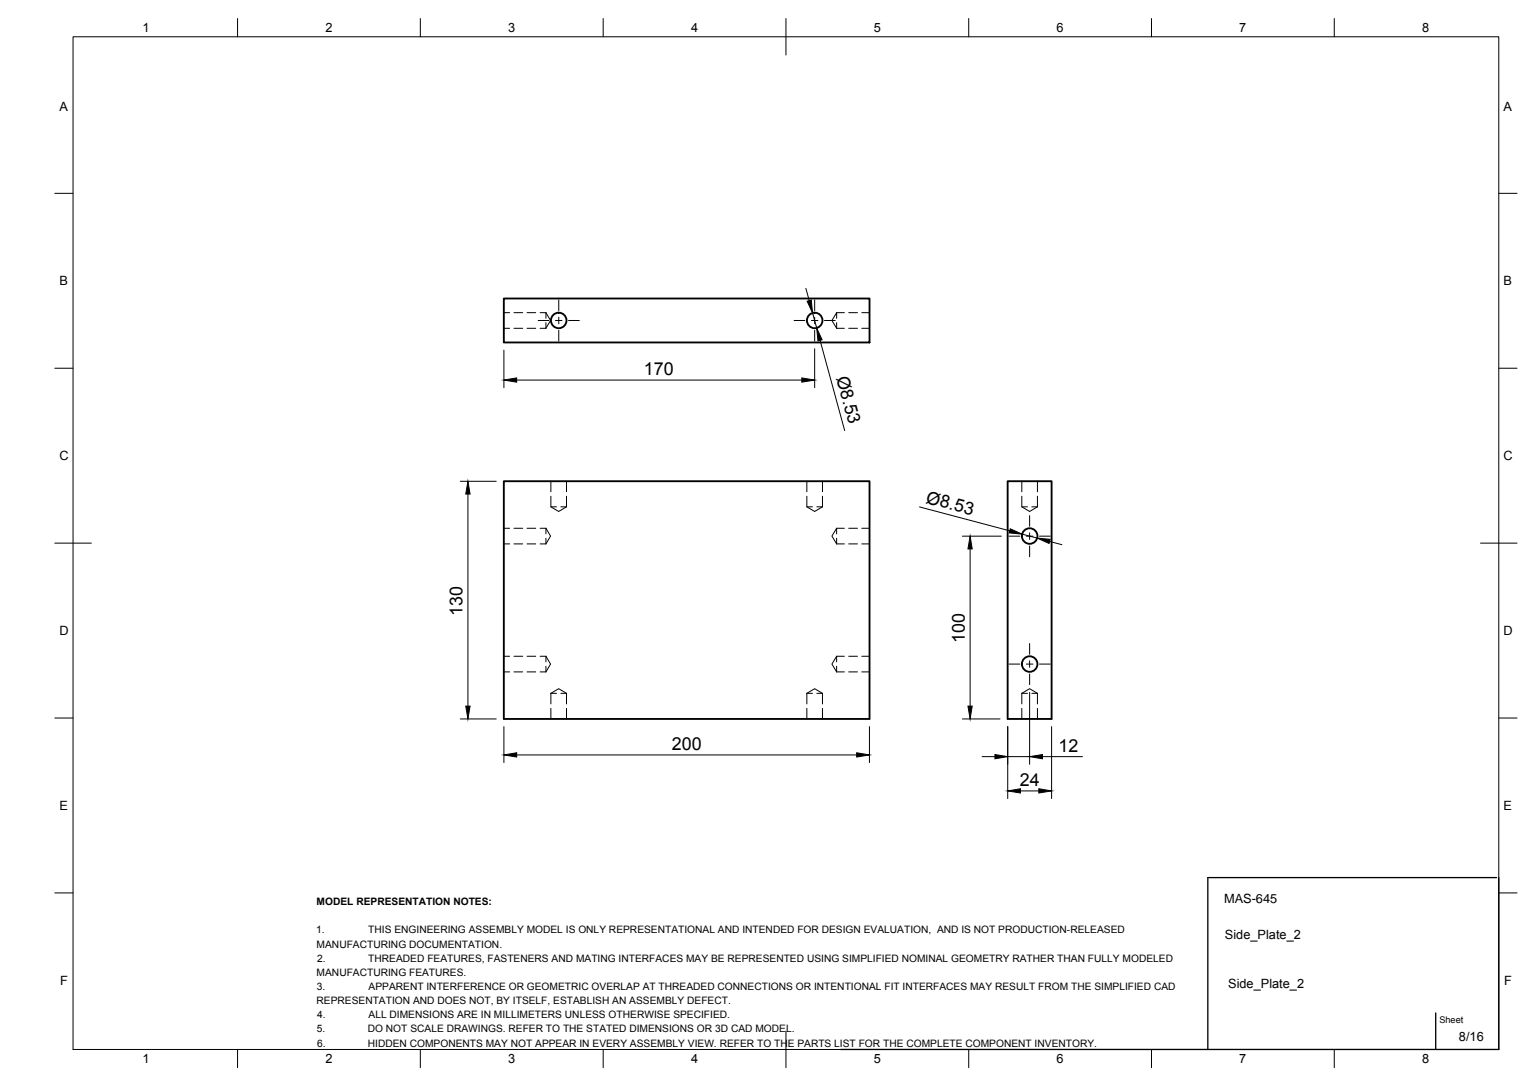
ISO-10303-21;
HEADER;
FILE_DESCRIPTION((''),'2;1');
FILE_NAME('Side_Plate_2.step','2026-10-09T10:54:55-07:00',(''),(''),'','','');
FILE_SCHEMA (('AUTOMOTIVE_DESIGN { 1 0 10303 214 3 1 1 }'));
ENDSEC;
DATA;
#10=MECHANICAL_DESIGN_GEOMETRIC_PRESENTATION_REPRESENTATION('',(#599),#63824);
#569=SHAPE_REPRESENTATION_RELATIONSHIP('SRR','None',#63883,#584) ;
#584=ADVANCED_BREP_SHAPE_REPRESENTATION('',(#614),#63813) ;
#599=STYLED_ITEM('',(#63963),#614) ;
#614=MANIFOLD_SOLID_BREP('Body1',#15498) ;
#723=FACE_BOUND('',#2671,.T.) ;
#724=FACE_BOUND('',#2672,.T.) ;
#725=FACE_BOUND('',#2679,.T.) ;
#726=FACE_BOUND('',#2680,.T.) ;
#727=FACE_BOUND('',#2683,.T.) ;
#728=FACE_BOUND('',#2684,.T.) ;
#729=FACE_BOUND('',#2686,.T.) ;
#730=FACE_BOUND('',#2687,.T.) ;
#876=PLANE('',#16011) ;
#877=PLANE('',#16020) ;
#878=PLANE('',#16021) ;
#879=PLANE('',#16022) ;
#880=PLANE('',#16023) ;
#881=PLANE('',#16024) ;
#1192=CYLINDRICAL_SURFACE('',#15989,4.263) ;
#1193=CYLINDRICAL_SURFACE('',#15993,4.263) ;
#1194=CYLINDRICAL_SURFACE('',#15997,4.263) ;
#1195=CYLINDRICAL_SURFACE('',#16001,4.263) ;
#1196=CYLINDRICAL_SURFACE('',#16005,4.263) ;
#1197=CYLINDRICAL_SURFACE('',#16009,4.263) ;
#1198=CYLINDRICAL_SURFACE('',#16014,4.263) ;
#1199=CYLINDRICAL_SURFACE('',#16018,4.263) ;
#1699=FACE_OUTER_BOUND('',#2658,.T.) ;
#1700=FACE_OUTER_BOUND('',#2659,.T.) ;
#1701=FACE_OUTER_BOUND('',#2660,.T.) ;
#1702=FACE_OUTER_BOUND('',#2661,.T.) ;
#1703=FACE_OUTER_BOUND('',#2662,.T.) ;
#1704=FACE_OUTER_BOUND('',#2663,.T.) ;
#1705=FACE_OUTER_BOUND('',#2664,.T.) ;
#1706=FACE_OUTER_BOUND('',#2665,.T.) ;
#1707=FACE_OUTER_BOUND('',#2666,.T.) ;
#1708=FACE_OUTER_BOUND('',#2667,.T.) ;
#1709=FACE_OUTER_BOUND('',#2668,.T.) ;
#1710=FACE_OUTER_BOUND('',#2669,.T.) ;
#1711=FACE_OUTER_BOUND('',#2670,.T.) ;
#1712=FACE_OUTER_BOUND('',#2673,.T.) ;
#1713=FACE_OUTER_BOUND('',#2674,.T.) ;
#1714=FACE_OUTER_BOUND('',#2675,.T.) ;
#1715=FACE_OUTER_BOUND('',#2676,.T.) ;
#1716=FACE_OUTER_BOUND('',#2677,.T.) ;
#1717=FACE_OUTER_BOUND('',#2678,.T.) ;
#1718=FACE_OUTER_BOUND('',#2681,.T.) ;
#1719=FACE_OUTER_BOUND('',#2682,.T.) ;
#1720=FACE_OUTER_BOUND('',#2685,.T.) ;
#2658=EDGE_LOOP('',(#10422,#10423,#10424)) ;
#2659=EDGE_LOOP('',(#10425,#10426,#10427,#10428)) ;
#2660=EDGE_LOOP('',(#10429,#10430,#10431)) ;
#2661=EDGE_LOOP('',(#10432,#10433,#10434,#10435)) ;
#2662=EDGE_LOOP('',(#10436,#10437,#10438)) ;
#2663=EDGE_LOOP('',(#10439,#10440,#10441,#10442)) ;
#2664=EDGE_LOOP('',(#10443,#10444,#10445)) ;
#2665=EDGE_LOOP('',(#10446,#10447,#10448,#10449)) ;
#2666=EDGE_LOOP('',(#10450,#10451,#10452)) ;
#2667=EDGE_LOOP('',(#10453,#10454,#10455,#10456)) ;
#2668=EDGE_LOOP('',(#10457,#10458,#10459)) ;
#2669=EDGE_LOOP('',(#10460,#10461,#10462,#10463)) ;
#2670=EDGE_LOOP('',(#10464,#10465,#10466,#10467)) ;
#2671=EDGE_LOOP('',(#10468)) ;
#2672=EDGE_LOOP('',(#10469)) ;
#2673=EDGE_LOOP('',(#10470,#10471,#10472)) ;
#2674=EDGE_LOOP('',(#10473,#10474,#10475,#10476)) ;
#2675=EDGE_LOOP('',(#10477,#10478,#10479)) ;
#2676=EDGE_LOOP('',(#10480,#10481,#10482,#10483)) ;
#2677=EDGE_LOOP('',(#10484,#10485,#10486,#10487)) ;
#2678=EDGE_LOOP('',(#10488,#10489,#10490,#10491)) ;
#2679=EDGE_LOOP('',(#10492)) ;
#2680=EDGE_LOOP('',(#10493)) ;
#2681=EDGE_LOOP('',(#10494,#10495,#10496,#10497)) ;
#2682=EDGE_LOOP('',(#10498,#10499,#10500,#10501)) ;
#2683=EDGE_LOOP('',(#10502)) ;
#2684=EDGE_LOOP('',(#10503)) ;
#2685=EDGE_LOOP('',(#10504,#10505,#10506,#10507)) ;
#2686=EDGE_LOOP('',(#10508)) ;
#2687=EDGE_LOOP('',(#10509)) ;
#3626=CIRCLE('',#15988,4.263) ;
#3627=CIRCLE('',#15990,4.263) ;
#3628=CIRCLE('',#15992,4.263) ;
#3629=CIRCLE('',#15994,4.263) ;
#3630=CIRCLE('',#15996,4.263) ;
#3631=CIRCLE('',#15998,4.263) ;
#3632=CIRCLE('',#16000,4.263) ;
#3633=CIRCLE('',#16002,4.263) ;
#3634=CIRCLE('',#16004,4.263) ;
#3635=CIRCLE('',#16006,4.263) ;
#3636=CIRCLE('',#16008,4.263) ;
#3637=CIRCLE('',#16010,4.263) ;
#3638=CIRCLE('',#16013,4.263) ;
#3639=CIRCLE('',#16015,4.263) ;
#3640=CIRCLE('',#16017,4.263) ;
#3641=CIRCLE('',#16019,4.263) ;
#4848=LINE('',#23703,#5504) ;
#4849=LINE('',#23708,#5505) ;
#4850=LINE('',#23712,#5506) ;
#4851=LINE('',#23717,#5507) ;
#4852=LINE('',#23721,#5508) ;
#4853=LINE('',#23726,#5509) ;
#4854=LINE('',#23730,#5510) ;
#4855=LINE('',#23735,#5511) ;
#4856=LINE('',#23739,#5512) ;
#4857=LINE('',#23744,#5513) ;
#4858=LINE('',#23748,#5514) ;
#4859=LINE('',#23753,#5515) ;
#4860=LINE('',#23757,#5516) ;
#4861=LINE('',#23759,#5517) ;
#4862=LINE('',#23761,#5518) ;
#4863=LINE('',#23762,#5519) ;
#4864=LINE('',#23766,#5520) ;
#4865=LINE('',#23770,#5521) ;
#4866=LINE('',#23775,#5522) ;
#4867=LINE('',#23779,#5523) ;
#4868=LINE('',#23784,#5524) ;
#4869=LINE('',#23785,#5525) ;
#4870=LINE('',#23786,#5526) ;
#4871=LINE('',#23789,#5527) ;
#4872=LINE('',#23790,#5528) ;
#4873=LINE('',#23793,#5529) ;
#4874=LINE('',#23794,#5530) ;
#4875=LINE('',#23796,#5531) ;
#5504=VECTOR('',#18686,2.42186816158307) ;
#5505=VECTOR('',#18693,4.263) ;
#5506=VECTOR('',#18696,2.42186816158307) ;
#5507=VECTOR('',#18703,4.263) ;
#5508=VECTOR('',#18706,2.42186816158307) ;
#5509=VECTOR('',#18713,4.263) ;
#5510=VECTOR('',#18716,2.42186816158307) ;
#5511=VECTOR('',#18723,4.263) ;
#5512=VECTOR('',#18726,2.42186816158307) ;
#5513=VECTOR('',#18733,4.263) ;
#5514=VECTOR('',#18736,2.42186816158307) ;
#5515=VECTOR('',#18743,4.263) ;
#5516=VECTOR('',#18746,10.) ;
#5517=VECTOR('',#18747,10.) ;
#5518=VECTOR('',#18748,10.) ;
#5519=VECTOR('',#18749,10.) ;
#5520=VECTOR('',#18752,2.42186816158307) ;
#5521=VECTOR('',#18757,4.263) ;
#5522=VECTOR('',#18762,2.42186816158307) ;
#5523=VECTOR('',#18767,4.263) ;
#5524=VECTOR('',#18772,10.) ;
#5525=VECTOR('',#18773,10.) ;
#5526=VECTOR('',#18774,10.) ;
#5527=VECTOR('',#18777,10.) ;
#5528=VECTOR('',#18778,10.) ;
#5529=VECTOR('',#18781,10.) ;
#5530=VECTOR('',#18782,10.) ;
#5531=VECTOR('',#18785,10.) ;
#6220=VERTEX_POINT('',#23701) ;
#6221=VERTEX_POINT('',#23702) ;
#6222=VERTEX_POINT('',#23706) ;
#6223=VERTEX_POINT('',#23710) ;
#6224=VERTEX_POINT('',#23711) ;
#6225=VERTEX_POINT('',#23715) ;
#6226=VERTEX_POINT('',#23719) ;
#6227=VERTEX_POINT('',#23720) ;
#6228=VERTEX_POINT('',#23724) ;
#6229=VERTEX_POINT('',#23728) ;
#6230=VERTEX_POINT('',#23729) ;
#6231=VERTEX_POINT('',#23733) ;
#6232=VERTEX_POINT('',#23737) ;
#6233=VERTEX_POINT('',#23738) ;
#6234=VERTEX_POINT('',#23742) ;
#6235=VERTEX_POINT('',#23746) ;
#6236=VERTEX_POINT('',#23747) ;
#6237=VERTEX_POINT('',#23751) ;
#6238=VERTEX_POINT('',#23755) ;
#6239=VERTEX_POINT('',#23756) ;
#6240=VERTEX_POINT('',#23758) ;
#6241=VERTEX_POINT('',#23760) ;
#6242=VERTEX_POINT('',#23764) ;
#6243=VERTEX_POINT('',#23765) ;
#6244=VERTEX_POINT('',#23769) ;
#6245=VERTEX_POINT('',#23773) ;
#6246=VERTEX_POINT('',#23774) ;
#6247=VERTEX_POINT('',#23778) ;
#6248=VERTEX_POINT('',#23782) ;
#6249=VERTEX_POINT('',#23783) ;
#6250=VERTEX_POINT('',#23788) ;
#6251=VERTEX_POINT('',#23792) ;
#7765=EDGE_CURVE('',#6220,#6221,#4848,.T.) ;
#7766=EDGE_CURVE('',#6221,#6221,#3626,.T.) ;
#7767=EDGE_CURVE('',#6222,#6222,#3627,.T.) ;
#7768=EDGE_CURVE('',#6222,#6221,#4849,.T.) ;
#7769=EDGE_CURVE('',#6223,#6224,#4850,.T.) ;
#7770=EDGE_CURVE('',#6224,#6224,#3628,.T.) ;
#7771=EDGE_CURVE('',#6225,#6225,#3629,.T.) ;
#7772=EDGE_CURVE('',#6225,#6224,#4851,.T.) ;
#7773=EDGE_CURVE('',#6226,#6227,#4852,.T.) ;
#7774=EDGE_CURVE('',#6227,#6227,#3630,.T.) ;
#7775=EDGE_CURVE('',#6228,#6228,#3631,.T.) ;
#7776=EDGE_CURVE('',#6228,#6227,#4853,.T.) ;
#7777=EDGE_CURVE('',#6229,#6230,#4854,.T.) ;
#7778=EDGE_CURVE('',#6230,#6230,#3632,.T.) ;
#7779=EDGE_CURVE('',#6231,#6231,#3633,.T.) ;
#7780=EDGE_CURVE('',#6231,#6230,#4855,.T.) ;
#7781=EDGE_CURVE('',#6232,#6233,#4856,.T.) ;
#7782=EDGE_CURVE('',#6233,#6233,#3634,.T.) ;
#7783=EDGE_CURVE('',#6234,#6234,#3635,.F.) ;
#7784=EDGE_CURVE('',#6234,#6233,#4857,.T.) ;
#7785=EDGE_CURVE('',#6235,#6236,#4858,.T.) ;
#7786=EDGE_CURVE('',#6236,#6236,#3636,.T.) ;
#7787=EDGE_CURVE('',#6237,#6237,#3637,.F.) ;
#7788=EDGE_CURVE('',#6237,#6236,#4859,.T.) ;
#7789=EDGE_CURVE('',#6238,#6239,#4860,.T.) ;
#7790=EDGE_CURVE('',#6239,#6240,#4861,.T.) ;
#7791=EDGE_CURVE('',#6240,#6241,#4862,.T.) ;
#7792=EDGE_CURVE('',#6241,#6238,#4863,.T.) ;
#7793=EDGE_CURVE('',#6242,#6243,#4864,.T.) ;
#7794=EDGE_CURVE('',#6243,#6243,#3638,.T.) ;
#7795=EDGE_CURVE('',#6243,#6244,#4865,.T.) ;
#7796=EDGE_CURVE('',#6244,#6244,#3639,.F.) ;
#7797=EDGE_CURVE('',#6245,#6246,#4866,.T.) ;
#7798=EDGE_CURVE('',#6246,#6246,#3640,.T.) ;
#7799=EDGE_CURVE('',#6246,#6247,#4867,.T.) ;
#7800=EDGE_CURVE('',#6247,#6247,#3641,.F.) ;
#7801=EDGE_CURVE('',#6248,#6249,#4868,.T.) ;
#7802=EDGE_CURVE('',#6249,#6240,#4869,.T.) ;
#7803=EDGE_CURVE('',#6248,#6239,#4870,.T.) ;
#7804=EDGE_CURVE('',#6249,#6250,#4871,.T.) ;
#7805=EDGE_CURVE('',#6250,#6241,#4872,.T.) ;
#7806=EDGE_CURVE('',#6250,#6251,#4873,.T.) ;
#7807=EDGE_CURVE('',#6251,#6238,#4874,.T.) ;
#7808=EDGE_CURVE('',#6251,#6248,#4875,.T.) ;
#10422=ORIENTED_EDGE('',*,*,#7765,.T.) ;
#10423=ORIENTED_EDGE('',*,*,#7766,.F.) ;
#10424=ORIENTED_EDGE('',*,*,#7765,.F.) ;
#10425=ORIENTED_EDGE('',*,*,#7767,.F.) ;
#10426=ORIENTED_EDGE('',*,*,#7768,.T.) ;
#10427=ORIENTED_EDGE('',*,*,#7766,.T.) ;
#10428=ORIENTED_EDGE('',*,*,#7768,.F.) ;
#10429=ORIENTED_EDGE('',*,*,#7769,.T.) ;
#10430=ORIENTED_EDGE('',*,*,#7770,.F.) ;
#10431=ORIENTED_EDGE('',*,*,#7769,.F.) ;
#10432=ORIENTED_EDGE('',*,*,#7771,.F.) ;
#10433=ORIENTED_EDGE('',*,*,#7772,.T.) ;
#10434=ORIENTED_EDGE('',*,*,#7770,.T.) ;
#10435=ORIENTED_EDGE('',*,*,#7772,.F.) ;
#10436=ORIENTED_EDGE('',*,*,#7773,.T.) ;
#10437=ORIENTED_EDGE('',*,*,#7774,.F.) ;
#10438=ORIENTED_EDGE('',*,*,#7773,.F.) ;
#10439=ORIENTED_EDGE('',*,*,#7775,.F.) ;
#10440=ORIENTED_EDGE('',*,*,#7776,.T.) ;
#10441=ORIENTED_EDGE('',*,*,#7774,.T.) ;
#10442=ORIENTED_EDGE('',*,*,#7776,.F.) ;
#10443=ORIENTED_EDGE('',*,*,#7777,.T.) ;
#10444=ORIENTED_EDGE('',*,*,#7778,.F.) ;
#10445=ORIENTED_EDGE('',*,*,#7777,.F.) ;
#10446=ORIENTED_EDGE('',*,*,#7779,.F.) ;
#10447=ORIENTED_EDGE('',*,*,#7780,.T.) ;
#10448=ORIENTED_EDGE('',*,*,#7778,.T.) ;
#10449=ORIENTED_EDGE('',*,*,#7780,.F.) ;
#10450=ORIENTED_EDGE('',*,*,#7781,.T.) ;
#10451=ORIENTED_EDGE('',*,*,#7782,.F.) ;
#10452=ORIENTED_EDGE('',*,*,#7781,.F.) ;
#10453=ORIENTED_EDGE('',*,*,#7783,.F.) ;
#10454=ORIENTED_EDGE('',*,*,#7784,.T.) ;
#10455=ORIENTED_EDGE('',*,*,#7782,.T.) ;
#10456=ORIENTED_EDGE('',*,*,#7784,.F.) ;
#10457=ORIENTED_EDGE('',*,*,#7785,.T.) ;
#10458=ORIENTED_EDGE('',*,*,#7786,.F.) ;
#10459=ORIENTED_EDGE('',*,*,#7785,.F.) ;
#10460=ORIENTED_EDGE('',*,*,#7787,.F.) ;
#10461=ORIENTED_EDGE('',*,*,#7788,.T.) ;
#10462=ORIENTED_EDGE('',*,*,#7786,.T.) ;
#10463=ORIENTED_EDGE('',*,*,#7788,.F.) ;
#10464=ORIENTED_EDGE('',*,*,#7789,.T.) ;
#10465=ORIENTED_EDGE('',*,*,#7790,.T.) ;
#10466=ORIENTED_EDGE('',*,*,#7791,.T.) ;
#10467=ORIENTED_EDGE('',*,*,#7792,.T.) ;
#10468=ORIENTED_EDGE('',*,*,#7783,.T.) ;
#10469=ORIENTED_EDGE('',*,*,#7787,.T.) ;
#10470=ORIENTED_EDGE('',*,*,#7793,.T.) ;
#10471=ORIENTED_EDGE('',*,*,#7794,.T.) ;
#10472=ORIENTED_EDGE('',*,*,#7793,.F.) ;
#10473=ORIENTED_EDGE('',*,*,#7794,.F.) ;
#10474=ORIENTED_EDGE('',*,*,#7795,.T.) ;
#10475=ORIENTED_EDGE('',*,*,#7796,.T.) ;
#10476=ORIENTED_EDGE('',*,*,#7795,.F.) ;
#10477=ORIENTED_EDGE('',*,*,#7797,.T.) ;
#10478=ORIENTED_EDGE('',*,*,#7798,.T.) ;
#10479=ORIENTED_EDGE('',*,*,#7797,.F.) ;
#10480=ORIENTED_EDGE('',*,*,#7798,.F.) ;
#10481=ORIENTED_EDGE('',*,*,#7799,.T.) ;
#10482=ORIENTED_EDGE('',*,*,#7800,.T.) ;
#10483=ORIENTED_EDGE('',*,*,#7799,.F.) ;
#10484=ORIENTED_EDGE('',*,*,#7801,.T.) ;
#10485=ORIENTED_EDGE('',*,*,#7802,.T.) ;
#10486=ORIENTED_EDGE('',*,*,#7790,.F.) ;
#10487=ORIENTED_EDGE('',*,*,#7803,.F.) ;
#10488=ORIENTED_EDGE('',*,*,#7804,.T.) ;
#10489=ORIENTED_EDGE('',*,*,#7805,.T.) ;
#10490=ORIENTED_EDGE('',*,*,#7791,.F.) ;
#10491=ORIENTED_EDGE('',*,*,#7802,.F.) ;
#10492=ORIENTED_EDGE('',*,*,#7767,.T.) ;
#10493=ORIENTED_EDGE('',*,*,#7771,.T.) ;
#10494=ORIENTED_EDGE('',*,*,#7806,.T.) ;
#10495=ORIENTED_EDGE('',*,*,#7807,.T.) ;
#10496=ORIENTED_EDGE('',*,*,#7792,.F.) ;
#10497=ORIENTED_EDGE('',*,*,#7805,.F.) ;
#10498=ORIENTED_EDGE('',*,*,#7808,.T.) ;
#10499=ORIENTED_EDGE('',*,*,#7803,.T.) ;
#10500=ORIENTED_EDGE('',*,*,#7789,.F.) ;
#10501=ORIENTED_EDGE('',*,*,#7807,.F.) ;
#10502=ORIENTED_EDGE('',*,*,#7775,.T.) ;
#10503=ORIENTED_EDGE('',*,*,#7779,.T.) ;
#10504=ORIENTED_EDGE('',*,*,#7808,.F.) ;
#10505=ORIENTED_EDGE('',*,*,#7806,.F.) ;
#10506=ORIENTED_EDGE('',*,*,#7804,.F.) ;
#10507=ORIENTED_EDGE('',*,*,#7801,.F.) ;
#10508=ORIENTED_EDGE('',*,*,#7796,.F.) ;
#10509=ORIENTED_EDGE('',*,*,#7800,.F.) ;
#14530=CONICAL_SURFACE('',#15987,2.42186816158307,1.02974425867665) ;
#14531=CONICAL_SURFACE('',#15991,2.42186816158307,1.02974425867665) ;
#14532=CONICAL_SURFACE('',#15995,2.42186816158307,1.02974425867665) ;
#14533=CONICAL_SURFACE('',#15999,2.42186816158307,1.02974425867665) ;
#14534=CONICAL_SURFACE('',#16003,2.42186816158307,1.02974425867665) ;
#14535=CONICAL_SURFACE('',#16007,2.42186816158307,1.02974425867665) ;
#14536=CONICAL_SURFACE('',#16012,2.42186816158307,1.02974425867665) ;
#14537=CONICAL_SURFACE('',#16016,2.42186816158307,1.02974425867665) ;
#14787=ADVANCED_FACE('',(#1699),#14530,.F.) ;
#14788=ADVANCED_FACE('',(#1700),#1192,.F.) ;
#14789=ADVANCED_FACE('',(#1701),#14531,.F.) ;
#14790=ADVANCED_FACE('',(#1702),#1193,.F.) ;
#14791=ADVANCED_FACE('',(#1703),#14532,.F.) ;
#14792=ADVANCED_FACE('',(#1704),#1194,.F.) ;
#14793=ADVANCED_FACE('',(#1705),#14533,.F.) ;
#14794=ADVANCED_FACE('',(#1706),#1195,.F.) ;
#14795=ADVANCED_FACE('',(#1707),#14534,.F.) ;
#14796=ADVANCED_FACE('',(#1708),#1196,.F.) ;
#14797=ADVANCED_FACE('',(#1709),#14535,.F.) ;
#14798=ADVANCED_FACE('',(#1710),#1197,.F.) ;
#14799=ADVANCED_FACE('',(#1711,#723,#724),#876,.F.) ;
#14800=ADVANCED_FACE('',(#1712),#14536,.F.) ;
#14801=ADVANCED_FACE('',(#1713),#1198,.F.) ;
#14802=ADVANCED_FACE('',(#1714),#14537,.F.) ;
#14803=ADVANCED_FACE('',(#1715),#1199,.F.) ;
#14804=ADVANCED_FACE('',(#1716),#877,.F.) ;
#14805=ADVANCED_FACE('',(#1717,#725,#726),#878,.F.) ;
#14806=ADVANCED_FACE('',(#1718),#879,.F.) ;
#14807=ADVANCED_FACE('',(#1719,#727,#728),#880,.F.) ;
#14808=ADVANCED_FACE('',(#1720,#729,#730),#881,.T.) ;
#15498=CLOSED_SHELL('',(#14787,#14788,#14789,#14790,#14791,#14792,#14793,
#14794,#14795,#14796,#14797,#14798,#14799,#14800,#14801,#14802,#14803,#14804,
#14805,#14806,#14807,#14808)) ;
#15986=AXIS2_PLACEMENT_3D('',#23699,#18682,#18683) ;
#15987=AXIS2_PLACEMENT_3D('',#23700,#18684,#18685) ;
#15988=AXIS2_PLACEMENT_3D('',#23704,#18687,#18688) ;
#15989=AXIS2_PLACEMENT_3D('',#23705,#18689,#18690) ;
#15990=AXIS2_PLACEMENT_3D('',#23707,#18691,#18692) ;
#15991=AXIS2_PLACEMENT_3D('',#23709,#18694,#18695) ;
#15992=AXIS2_PLACEMENT_3D('',#23713,#18697,#18698) ;
#15993=AXIS2_PLACEMENT_3D('',#23714,#18699,#18700) ;
#15994=AXIS2_PLACEMENT_3D('',#23716,#18701,#18702) ;
#15995=AXIS2_PLACEMENT_3D('',#23718,#18704,#18705) ;
#15996=AXIS2_PLACEMENT_3D('',#23722,#18707,#18708) ;
#15997=AXIS2_PLACEMENT_3D('',#23723,#18709,#18710) ;
#15998=AXIS2_PLACEMENT_3D('',#23725,#18711,#18712) ;
#15999=AXIS2_PLACEMENT_3D('',#23727,#18714,#18715) ;
#16000=AXIS2_PLACEMENT_3D('',#23731,#18717,#18718) ;
#16001=AXIS2_PLACEMENT_3D('',#23732,#18719,#18720) ;
#16002=AXIS2_PLACEMENT_3D('',#23734,#18721,#18722) ;
#16003=AXIS2_PLACEMENT_3D('',#23736,#18724,#18725) ;
#16004=AXIS2_PLACEMENT_3D('',#23740,#18727,#18728) ;
#16005=AXIS2_PLACEMENT_3D('',#23741,#18729,#18730) ;
#16006=AXIS2_PLACEMENT_3D('',#23743,#18731,#18732) ;
#16007=AXIS2_PLACEMENT_3D('',#23745,#18734,#18735) ;
#16008=AXIS2_PLACEMENT_3D('',#23749,#18737,#18738) ;
#16009=AXIS2_PLACEMENT_3D('',#23750,#18739,#18740) ;
#16010=AXIS2_PLACEMENT_3D('',#23752,#18741,#18742) ;
#16011=AXIS2_PLACEMENT_3D('',#23754,#18744,#18745) ;
#16012=AXIS2_PLACEMENT_3D('',#23763,#18750,#18751) ;
#16013=AXIS2_PLACEMENT_3D('',#23767,#18753,#18754) ;
#16014=AXIS2_PLACEMENT_3D('',#23768,#18755,#18756) ;
#16015=AXIS2_PLACEMENT_3D('',#23771,#18758,#18759) ;
#16016=AXIS2_PLACEMENT_3D('',#23772,#18760,#18761) ;
#16017=AXIS2_PLACEMENT_3D('',#23776,#18763,#18764) ;
#16018=AXIS2_PLACEMENT_3D('',#23777,#18765,#18766) ;
#16019=AXIS2_PLACEMENT_3D('',#23780,#18768,#18769) ;
#16020=AXIS2_PLACEMENT_3D('',#23781,#18770,#18771) ;
#16021=AXIS2_PLACEMENT_3D('',#23787,#18775,#18776) ;
#16022=AXIS2_PLACEMENT_3D('',#23791,#18779,#18780) ;
#16023=AXIS2_PLACEMENT_3D('',#23795,#18783,#18784) ;
#16024=AXIS2_PLACEMENT_3D('',#23797,#18786,#18787) ;
#18682=DIRECTION('axis',(0.,0.,1.)) ;
#18683=DIRECTION('refdir',(1.,0.,0.)) ;
#18684=DIRECTION('center_axis',(9.473903143468E-16,1.,0.)) ;
#18685=DIRECTION('ref_axis',(0.,0.,-1.)) ;
#18686=DIRECTION('',(5.92914802803472E-16,0.515038074910058,0.85716730070211)) ;
#18687=DIRECTION('center_axis',(-9.473903143468E-16,-1.,0.)) ;
#18688=DIRECTION('ref_axis',(0.,0.,-1.)) ;
#18689=DIRECTION('center_axis',(-9.473903143468E-16,-1.,0.)) ;
#18690=DIRECTION('ref_axis',(0.,0.,-1.)) ;
#18691=DIRECTION('center_axis',(9.47390314346801E-16,-1.,0.)) ;
#18692=DIRECTION('ref_axis',(0.,0.,-1.)) ;
#18693=DIRECTION('',(-9.473903143468E-16,-1.,0.)) ;
#18694=DIRECTION('center_axis',(9.473903143468E-16,1.,0.)) ;
#18695=DIRECTION('ref_axis',(0.,0.,-1.)) ;
#18696=DIRECTION('',(5.92914802803472E-16,0.515038074910058,0.85716730070211)) ;
#18697=DIRECTION('center_axis',(-9.473903143468E-16,-1.,0.)) ;
#18698=DIRECTION('ref_axis',(0.,0.,-1.)) ;
#18699=DIRECTION('center_axis',(-9.473903143468E-16,-1.,0.)) ;
#18700=DIRECTION('ref_axis',(0.,0.,-1.)) ;
#18701=DIRECTION('center_axis',(9.47390314346801E-16,-1.,0.)) ;
#18702=DIRECTION('ref_axis',(0.,0.,-1.)) ;
#18703=DIRECTION('',(-9.473903143468E-16,-1.,0.)) ;
#18704=DIRECTION('center_axis',(3.5527136788005E-16,-1.,0.)) ;
#18705=DIRECTION('ref_axis',(0.,0.,1.)) ;
#18706=DIRECTION('',(2.87951000497466E-16,-0.515038074910058,-0.85716730070211)) ;
#18707=DIRECTION('center_axis',(-3.5527136788005E-16,1.,0.)) ;
#18708=DIRECTION('ref_axis',(0.,0.,1.)) ;
#18709=DIRECTION('center_axis',(-3.5527136788005E-16,1.,0.)) ;
#18710=DIRECTION('ref_axis',(0.,0.,1.)) ;
#18711=DIRECTION('center_axis',(4.2632564145606E-15,1.,0.)) ;
#18712=DIRECTION('ref_axis',(0.,0.,1.)) ;
#18713=DIRECTION('',(-3.5527136788005E-16,1.,0.)) ;
#18714=DIRECTION('center_axis',(3.5527136788005E-16,-1.,0.)) ;
#18715=DIRECTION('ref_axis',(0.,0.,1.)) ;
#18716=DIRECTION('',(2.87951000497466E-16,-0.515038074910058,-0.85716730070211)) ;
#18717=DIRECTION('center_axis',(-3.5527136788005E-16,1.,0.)) ;
#18718=DIRECTION('ref_axis',(0.,0.,1.)) ;
#18719=DIRECTION('center_axis',(-3.5527136788005E-16,1.,0.)) ;
#18720=DIRECTION('ref_axis',(0.,0.,1.)) ;
#18721=DIRECTION('center_axis',(4.2632564145606E-15,1.,0.)) ;
#18722=DIRECTION('ref_axis',(0.,0.,1.)) ;
#18723=DIRECTION('',(-3.5527136788005E-16,1.,0.)) ;
#18724=DIRECTION('center_axis',(0.,0.,1.)) ;
#18725=DIRECTION('ref_axis',(1.,0.,0.)) ;
#18726=DIRECTION('',(-0.85716730070211,-1.04972719113862E-16,0.515038074910058)) ;
#18727=DIRECTION('center_axis',(0.,0.,-1.)) ;
#18728=DIRECTION('ref_axis',(1.,0.,0.)) ;
#18729=DIRECTION('center_axis',(0.,0.,-1.)) ;
#18730=DIRECTION('ref_axis',(1.,0.,0.)) ;
#18731=DIRECTION('center_axis',(0.,0.,1.)) ;
#18732=DIRECTION('ref_axis',(1.,0.,0.)) ;
#18733=DIRECTION('',(0.,0.,-1.)) ;
#18734=DIRECTION('center_axis',(0.,0.,1.)) ;
#18735=DIRECTION('ref_axis',(1.,0.,0.)) ;
#18736=DIRECTION('',(-0.85716730070211,-1.04972719113862E-16,0.515038074910058)) ;
#18737=DIRECTION('center_axis',(0.,0.,-1.)) ;
#18738=DIRECTION('ref_axis',(1.,0.,0.)) ;
#18739=DIRECTION('center_axis',(0.,0.,-1.)) ;
#18740=DIRECTION('ref_axis',(1.,0.,0.)) ;
#18741=DIRECTION('center_axis',(0.,0.,1.)) ;
#18742=DIRECTION('ref_axis',(1.,0.,0.)) ;
#18743=DIRECTION('',(0.,0.,-1.)) ;
#18744=DIRECTION('center_axis',(0.,0.,-1.)) ;
#18745=DIRECTION('ref_axis',(-1.,0.,0.)) ;
#18746=DIRECTION('',(1.,-4.2632564145606E-15,0.)) ;
#18747=DIRECTION('',(2.66453525910036E-16,1.,0.)) ;
#18748=DIRECTION('',(-1.,-9.47390314346801E-16,0.)) ;
#18749=DIRECTION('',(1.02140518265514E-15,-1.,0.)) ;
#18750=DIRECTION('center_axis',(0.,0.,-1.)) ;
#18751=DIRECTION('ref_axis',(1.,0.,0.)) ;
#18752=DIRECTION('',(-0.85716730070211,1.04972719113862E-16,-0.515038074910058)) ;
#18753=DIRECTION('center_axis',(0.,0.,-1.)) ;
#18754=DIRECTION('ref_axis',(1.,0.,0.)) ;
#18755=DIRECTION('center_axis',(0.,0.,-1.)) ;
#18756=DIRECTION('ref_axis',(1.,0.,0.)) ;
#18757=DIRECTION('',(0.,0.,-1.)) ;
#18758=DIRECTION('center_axis',(0.,0.,1.)) ;
#18759=DIRECTION('ref_axis',(1.,0.,0.)) ;
#18760=DIRECTION('center_axis',(0.,0.,-1.)) ;
#18761=DIRECTION('ref_axis',(1.,0.,0.)) ;
#18762=DIRECTION('',(-0.85716730070211,1.04972719113862E-16,-0.515038074910058)) ;
#18763=DIRECTION('center_axis',(0.,0.,-1.)) ;
#18764=DIRECTION('ref_axis',(1.,0.,0.)) ;
#18765=DIRECTION('center_axis',(0.,0.,-1.)) ;
#18766=DIRECTION('ref_axis',(1.,0.,0.)) ;
#18767=DIRECTION('',(0.,0.,-1.)) ;
#18768=DIRECTION('center_axis',(0.,0.,1.)) ;
#18769=DIRECTION('ref_axis',(1.,0.,0.)) ;
#18770=DIRECTION('center_axis',(-1.,2.66453525910036E-16,0.)) ;
#18771=DIRECTION('ref_axis',(-2.66453525910036E-16,-1.,0.)) ;
#18772=DIRECTION('',(2.66453525910036E-16,1.,0.)) ;
#18773=DIRECTION('',(0.,0.,1.)) ;
#18774=DIRECTION('',(0.,0.,1.)) ;
#18775=DIRECTION('center_axis',(9.47390314346801E-16,-1.,0.)) ;
#18776=DIRECTION('ref_axis',(1.,9.47390314346801E-16,0.)) ;
#18777=DIRECTION('',(-1.,-9.47390314346801E-16,0.)) ;
#18778=DIRECTION('',(0.,0.,1.)) ;
#18779=DIRECTION('center_axis',(1.,1.02140518265514E-15,0.)) ;
#18780=DIRECTION('ref_axis',(-1.02140518265514E-15,1.,0.)) ;
#18781=DIRECTION('',(1.02140518265514E-15,-1.,0.)) ;
#18782=DIRECTION('',(0.,0.,1.)) ;
#18783=DIRECTION('center_axis',(4.2632564145606E-15,1.,0.)) ;
#18784=DIRECTION('ref_axis',(-1.,4.2632564145606E-15,0.)) ;
#18785=DIRECTION('',(1.,-4.2632564145606E-15,0.)) ;
#18786=DIRECTION('center_axis',(0.,0.,-1.)) ;
#18787=DIRECTION('ref_axis',(-1.,0.,0.)) ;
#23699=CARTESIAN_POINT('',(0.,0.,0.)) ;
#23700=CARTESIAN_POINT('Origin',(63.0000000000011,385.343736383857,54.)) ;
#23701=CARTESIAN_POINT('',(63.0000000000011,383.888531181086,54.)) ;
#23702=CARTESIAN_POINT('',(63.0000000000011,386.45,58.263)) ;
#23703=CARTESIAN_POINT('',(63.0000000000011,385.343736383857,56.4218681615831)) ;
#23704=CARTESIAN_POINT('Origin',(63.0000000000011,386.45,54.)) ;
#23705=CARTESIAN_POINT('Origin',(63.0000000000011,405.45,54.)) ;
#23706=CARTESIAN_POINT('',(63.0000000000011,409.45,58.263)) ;
#23707=CARTESIAN_POINT('Origin',(63.0000000000011,409.45,54.)) ;
#23708=CARTESIAN_POINT('',(63.0000000000011,405.45,58.263)) ;
#23709=CARTESIAN_POINT('Origin',(63.0000000000011,385.343736383857,124.)) ;
#23710=CARTESIAN_POINT('',(63.0000000000011,383.888531181086,124.)) ;
#23711=CARTESIAN_POINT('',(63.0000000000011,386.45,128.263)) ;
#23712=CARTESIAN_POINT('',(63.0000000000011,385.343736383857,126.421868161583)) ;
#23713=CARTESIAN_POINT('Origin',(63.0000000000011,386.45,124.)) ;
#23714=CARTESIAN_POINT('Origin',(63.0000000000011,405.45,124.)) ;
#23715=CARTESIAN_POINT('',(63.0000000000011,409.45,128.263)) ;
#23716=CARTESIAN_POINT('Origin',(63.0000000000011,409.45,124.)) ;
#23717=CARTESIAN_POINT('',(63.0000000000011,405.45,128.263)) ;
#23718=CARTESIAN_POINT('Origin',(63.0000000000005,228.556263616143,124.)) ;
#23719=CARTESIAN_POINT('',(63.0000000000005,230.011468818915,124.)) ;
#23720=CARTESIAN_POINT('',(63.0000000000005,227.45,119.737)) ;
#23721=CARTESIAN_POINT('',(63.0000000000005,228.556263616143,121.578131838417)) ;
#23722=CARTESIAN_POINT('Origin',(63.0000000000005,227.45,124.)) ;
#23723=CARTESIAN_POINT('Origin',(63.0000000000005,208.45,124.)) ;
#23724=CARTESIAN_POINT('',(63.0000000000005,209.449999999999,119.737)) ;
#23725=CARTESIAN_POINT('Origin',(63.0000000000005,209.449999999999,124.)) ;
#23726=CARTESIAN_POINT('',(63.0000000000005,208.45,119.737)) ;
#23727=CARTESIAN_POINT('Origin',(63.0000000000005,228.556263616143,54.)) ;
#23728=CARTESIAN_POINT('',(63.0000000000005,230.011468818915,54.)) ;
#23729=CARTESIAN_POINT('',(63.0000000000005,227.45,49.737)) ;
#23730=CARTESIAN_POINT('',(63.0000000000005,228.556263616143,51.5781318384169)) ;
#23731=CARTESIAN_POINT('Origin',(63.0000000000005,227.45,54.)) ;
#23732=CARTESIAN_POINT('Origin',(63.0000000000005,208.45,54.)) ;
#23733=CARTESIAN_POINT('',(63.0000000000005,209.449999999999,49.737)) ;
#23734=CARTESIAN_POINT('Origin',(63.0000000000005,209.449999999999,54.)) ;
#23735=CARTESIAN_POINT('',(63.0000000000005,208.45,49.737)) ;
#23736=CARTESIAN_POINT('Origin',(63.,379.45,138.893736383857)) ;
#23737=CARTESIAN_POINT('',(63.,379.45,137.438531181086)) ;
#23738=CARTESIAN_POINT('',(58.737,379.45,140.)) ;
#23739=CARTESIAN_POINT('',(60.5781318384169,379.45,138.893736383857)) ;
#23740=CARTESIAN_POINT('Origin',(63.,379.45,140.)) ;
#23741=CARTESIAN_POINT('Origin',(63.,379.45,159.)) ;
#23742=CARTESIAN_POINT('',(58.737,379.45,154.)) ;
#23743=CARTESIAN_POINT('Origin',(63.,379.45,154.)) ;
#23744=CARTESIAN_POINT('',(58.737,379.45,159.)) ;
#23745=CARTESIAN_POINT('Origin',(63.,239.45,138.893736383857)) ;
#23746=CARTESIAN_POINT('',(63.,239.45,137.438531181086)) ;
#23747=CARTESIAN_POINT('',(58.737,239.45,140.)) ;
#23748=CARTESIAN_POINT('',(60.5781318384169,239.45,138.893736383857)) ;
#23749=CARTESIAN_POINT('Origin',(63.,239.45,140.)) ;
#23750=CARTESIAN_POINT('Origin',(63.,239.45,159.)) ;
#23751=CARTESIAN_POINT('',(58.737,239.45,154.)) ;
#23752=CARTESIAN_POINT('Origin',(63.,239.45,154.)) ;
#23753=CARTESIAN_POINT('',(58.737,239.45,159.)) ;
#23754=CARTESIAN_POINT('Origin',(63.,309.45,154.)) ;
#23755=CARTESIAN_POINT('',(51.0000000000001,209.449999999999,154.)) ;
#23756=CARTESIAN_POINT('',(75.,209.449999999999,154.)) ;
#23757=CARTESIAN_POINT('',(68.9999999999998,209.449999999999,154.)) ;
#23758=CARTESIAN_POINT('',(75.0000000000001,409.45,154.)) ;
#23759=CARTESIAN_POINT('',(75.0000000000001,359.45,154.)) ;
#23760=CARTESIAN_POINT('',(50.9999999999999,409.45,154.)) ;
#23761=CARTESIAN_POINT('',(56.9999999999999,409.45,154.)) ;
#23762=CARTESIAN_POINT('',(51.0000000000001,259.449999999999,154.)) ;
#23763=CARTESIAN_POINT('Origin',(63.,379.45,39.1062636161425)) ;
#23764=CARTESIAN_POINT('',(63.,379.45,40.5614688189145)) ;
#23765=CARTESIAN_POINT('',(58.737,379.45,38.)) ;
#23766=CARTESIAN_POINT('',(60.5781318384169,379.45,39.1062636161425)) ;
#23767=CARTESIAN_POINT('Origin',(63.,379.45,38.)) ;
#23768=CARTESIAN_POINT('Origin',(63.,379.45,19.)) ;
#23769=CARTESIAN_POINT('',(58.737,379.45,24.)) ;
#23770=CARTESIAN_POINT('',(58.737,379.45,19.)) ;
#23771=CARTESIAN_POINT('Origin',(63.,379.45,24.)) ;
#23772=CARTESIAN_POINT('Origin',(63.,239.45,39.1062636161425)) ;
#23773=CARTESIAN_POINT('',(63.,239.45,40.5614688189145)) ;
#23774=CARTESIAN_POINT('',(58.737,239.45,38.)) ;
#23775=CARTESIAN_POINT('',(60.5781318384169,239.45,39.1062636161425)) ;
#23776=CARTESIAN_POINT('Origin',(63.,239.45,38.)) ;
#23777=CARTESIAN_POINT('Origin',(63.,239.45,19.)) ;
#23778=CARTESIAN_POINT('',(58.737,239.45,24.)) ;
#23779=CARTESIAN_POINT('',(58.737,239.45,19.)) ;
#23780=CARTESIAN_POINT('Origin',(63.,239.45,24.)) ;
#23781=CARTESIAN_POINT('Origin',(75.0000000000001,409.45,24.)) ;
#23782=CARTESIAN_POINT('',(75.,209.449999999999,24.)) ;
#23783=CARTESIAN_POINT('',(75.0000000000001,409.45,24.)) ;
#23784=CARTESIAN_POINT('',(75.0000000000001,359.45,24.)) ;
#23785=CARTESIAN_POINT('',(75.0000000000001,409.45,24.)) ;
#23786=CARTESIAN_POINT('',(75.,209.449999999999,24.)) ;
#23787=CARTESIAN_POINT('Origin',(50.9999999999999,409.45,24.)) ;
#23788=CARTESIAN_POINT('',(50.9999999999999,409.45,24.)) ;
#23789=CARTESIAN_POINT('',(56.9999999999999,409.45,24.)) ;
#23790=CARTESIAN_POINT('',(50.9999999999999,409.45,24.)) ;
#23791=CARTESIAN_POINT('Origin',(51.0000000000001,209.449999999999,24.)) ;
#23792=CARTESIAN_POINT('',(51.0000000000001,209.449999999999,24.)) ;
#23793=CARTESIAN_POINT('',(51.0000000000001,259.449999999999,24.)) ;
#23794=CARTESIAN_POINT('',(51.0000000000001,209.449999999999,24.)) ;
#23795=CARTESIAN_POINT('Origin',(75.,209.449999999999,24.)) ;
#23796=CARTESIAN_POINT('',(68.9999999999998,209.449999999999,24.)) ;
#23797=CARTESIAN_POINT('Origin',(63.,309.45,24.)) ;
#63796=UNCERTAINTY_MEASURE_WITH_UNIT(LENGTH_MEASURE(0.01),#63825,
'DISTANCE_ACCURACY_VALUE',
'Maximum model space distance between geometric entities at asserted c
onnectivities') ;
#63807=UNCERTAINTY_MEASURE_WITH_UNIT(LENGTH_MEASURE(0.01),#63825,
'DISTANCE_ACCURACY_VALUE',
'Maximum model space distance between geometric entities at asserted c
onnectivities') ;
#63813=(
GEOMETRIC_REPRESENTATION_CONTEXT(3)
GLOBAL_UNCERTAINTY_ASSIGNED_CONTEXT((#63796))
GLOBAL_UNIT_ASSIGNED_CONTEXT((#63825,#63827,#63828))
REPRESENTATION_CONTEXT('','3D')
) ;
#63824=(
GEOMETRIC_REPRESENTATION_CONTEXT(3)
GLOBAL_UNCERTAINTY_ASSIGNED_CONTEXT((#63807))
GLOBAL_UNIT_ASSIGNED_CONTEXT((#63825,#63827,#63828))
REPRESENTATION_CONTEXT('','3D')
) ;
#63825=(
LENGTH_UNIT()
NAMED_UNIT(*)
SI_UNIT(.MILLI.,.METRE.)
) ;
#63827=(
NAMED_UNIT(*)
PLANE_ANGLE_UNIT()
SI_UNIT($,.RADIAN.)
) ;
#63828=(
NAMED_UNIT(*)
SI_UNIT($,.STERADIAN.)
SOLID_ANGLE_UNIT()
) ;
#63834=SHAPE_DEFINITION_REPRESENTATION(#63850,#63883) ;
#63850=PRODUCT_DEFINITION_SHAPE('',$,#63900) ;
#63883=SHAPE_REPRESENTATION('',(#15986),#63813) ;
#63894=PRODUCT_DEFINITION_CONTEXT('part definition',#63944,'design') ;
#63900=PRODUCT_DEFINITION('Side_Plate_2','Side_Plate_2',#63916,#63894) ;
#63916=PRODUCT_DEFINITION_FORMATION('',$,#63951) ;
#63944=APPLICATION_CONTEXT(
'Core Data for Automotive Mechanical Design Process') ;
#63945=PRODUCT_CONTEXT('part definition',#63944,'mechanical') ;
#63951=PRODUCT('Side_Plate_2','Side_Plate_2',$,(#63945)) ;
#63963=PRESENTATION_STYLE_ASSIGNMENT((#63968)) ;
#63968=SURFACE_STYLE_USAGE(.BOTH.,#63973) ;
#63973=SURFACE_SIDE_STYLE('',(#63978)) ;
#63978=SURFACE_STYLE_FILL_AREA(#63983) ;
#63983=FILL_AREA_STYLE('Opaque(160,160,160)',(#63988)) ;
#63988=FILL_AREA_STYLE_COLOUR('Opaque(160,160,160)',#63993) ;
#63993=COLOUR_RGB('Opaque(160,160,160)', 0.09019608, 0.27058824, 0.51372549) ;
ENDSEC;
END-ISO-10303-21;
